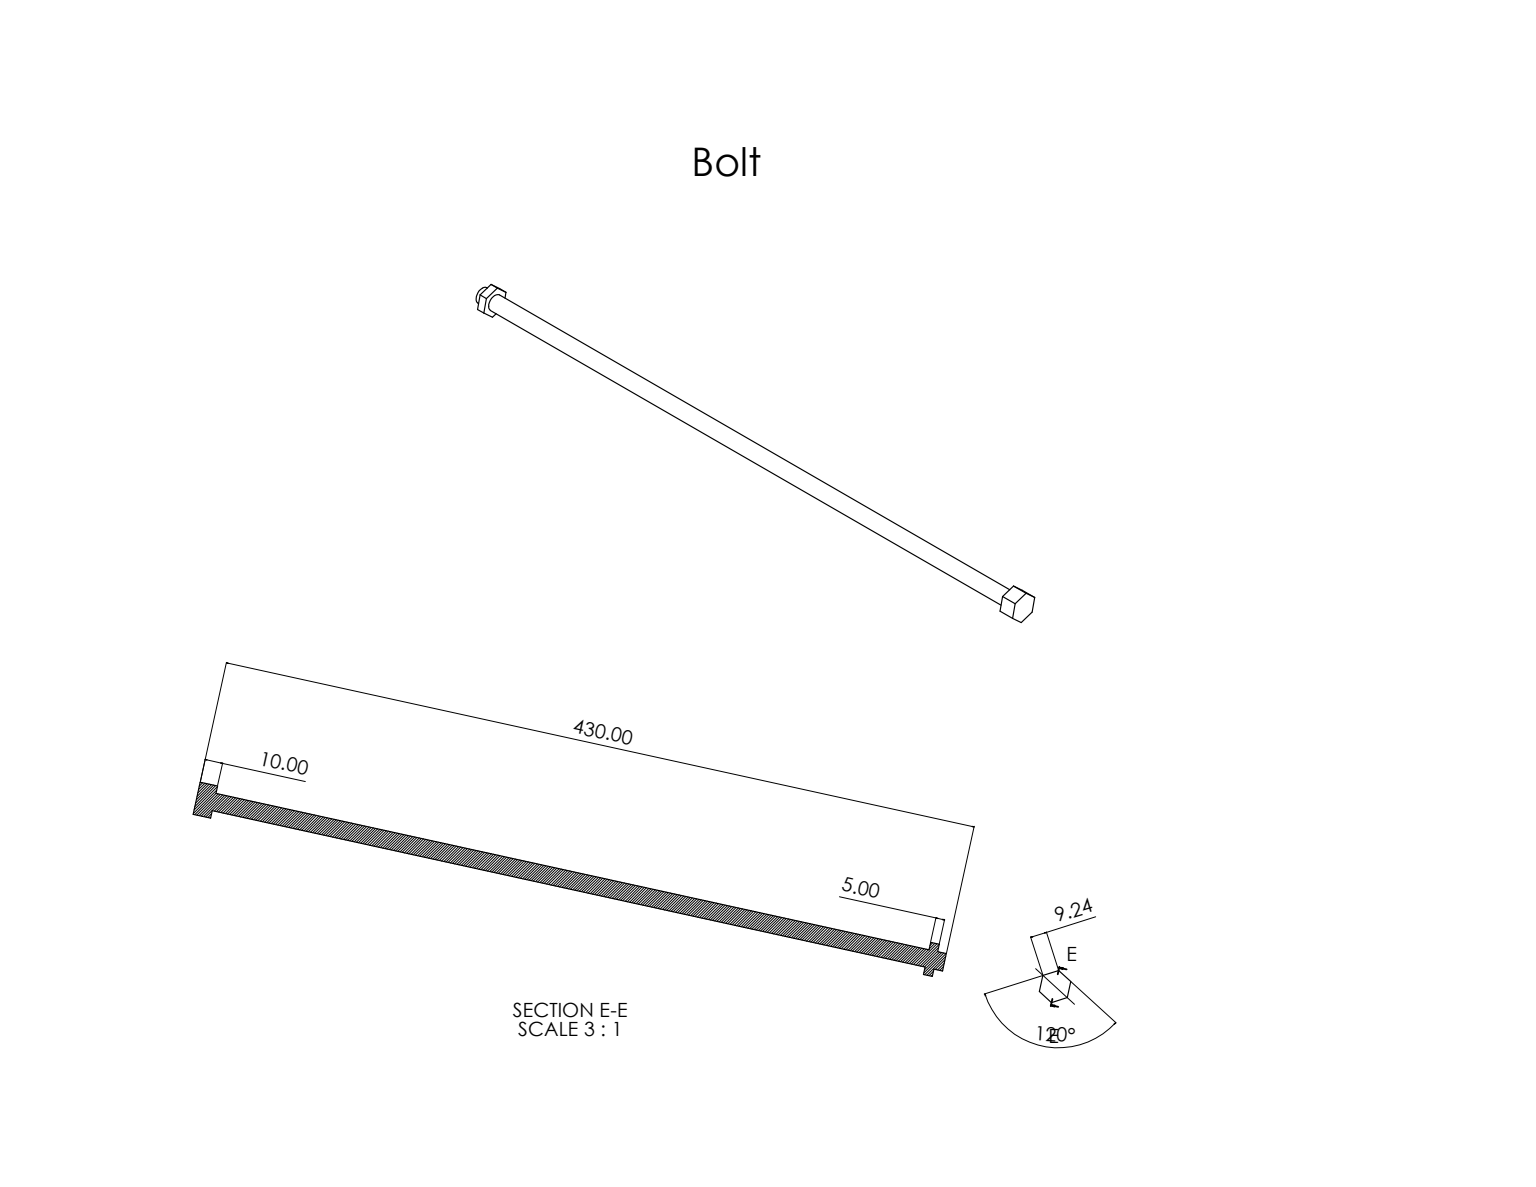
ISO-10303-21;
HEADER;
FILE_DESCRIPTION (('STEP AP214'),
    '1' );
FILE_NAME ('Bolt.step',
    '2026-10-27T19:20:31',
    ( '' ),
    ( '' ),
    'SwSTEP 2.0',
    'SolidWorks 2025',
    '' );
FILE_SCHEMA (( 'AUTOMOTIVE_DESIGN' ));
ENDSEC;

DATA;
#7=DIRECTION ( 'NONE',  ( 0.000000000000000000, 0.000000000000000000, -1.000000000000000000 ) ) ;
#22=DIRECTION ( 'NONE',  ( 0.000000000000000000, 0.000000000000000000, 1.000000000000000000 ) ) ;
#49=EDGE_CURVE ( 'NONE', #17928, #4130, #15424, .T. ) ;
#84=AXIS2_PLACEMENT_3D ( 'NONE', #861, #18677, #15078 ) ;
#112=ORIENTED_EDGE ( 'NONE', *, *, #21174, .F. ) ;
#117=EDGE_CURVE ( 'NONE', #6149, #16510, #26225, .T. ) ;
#141=ADVANCED_FACE ( 'NONE', ( #24347 ), #25952, .T. ) ;
#186=ORIENTED_EDGE ( 'NONE', *, *, #13817, .T. ) ;
#194=DIRECTION ( 'NONE',  ( 0.000000000000000000, -0.9767746502210199466, 0.2142691827715878239 ) ) ;
#196=CARTESIAN_POINT ( 'NONE',  ( 210.0000000000000284, 61.50000000000009948, -66.50000000000005684 ) ) ;
#258=PLANE ( 'NONE',  #2201 ) ;
#310=DIRECTION ( 'NONE',  ( 0.000000000000000000, -0.6739498806388346530, -0.7387770694782699321 ) ) ;
#394=ORIENTED_EDGE ( 'NONE', *, *, #6967, .F. ) ;
#426=( NAMED_UNIT ( * ) SI_UNIT ( $, .STERADIAN. ) SOLID_ANGLE_UNIT ( ) );
#446=DIRECTION ( 'NONE',  ( 0.000000000000000000, 0.000000000000000000, -1.000000000000000000 ) ) ;
#471=CARTESIAN_POINT ( 'NONE',  ( -215.0000000000000284, 69.29737539576900929, -75.30386416458597409 ) ) ;
#528=ORIENTED_EDGE ( 'NONE', *, *, #7839, .T. ) ;
#540=CARTESIAN_POINT ( 'NONE',  ( -215.0000000000000284, 61.50000000000001421, -66.50000000000005684 ) ) ;
#553=CARTESIAN_POINT ( 'NONE',  ( -210.0000000000000284, 72.72568232011437317, -59.67546976104961942 ) ) ;
#556=DIRECTION ( 'NONE',  ( -1.000000000000000000, -1.836970198721030427E-16, 0.000000000000000000 ) ) ;
#568=ORIENTED_EDGE ( 'NONE', *, *, #18157, .T. ) ;
#576=FACE_OUTER_BOUND ( 'NONE', #10089, .T. ) ;
#580=LINE ( 'NONE', #4839, #17878 ) ;
#732=DIRECTION ( 'NONE',  ( 1.000000000000000000, 1.836970198721030181E-16, 0.000000000000000000 ) ) ;
#831=EDGE_LOOP ( 'NONE', ( #23466, #9560, #14259, #11065 ) ) ;
#861=CARTESIAN_POINT ( 'NONE',  ( 200.0000000000000000, 66.50000000000009948, -66.50000000000005684 ) ) ;
#876=LINE ( 'NONE', #6848, #22484 ) ;
#879=CARTESIAN_POINT ( 'NONE',  ( 210.0000000000000284, 69.29737539576909455, -75.30386416458597409 ) ) ;
#902=CARTESIAN_POINT ( 'NONE',  ( 210.0000000000000284, 72.72568232011447265, -59.67546976104962653 ) ) ;
#912=CARTESIAN_POINT ( 'NONE',  ( -210.0000000000000284, 63.70262460423102624, -57.69613583541415380 ) ) ;
#916=VERTEX_POINT ( 'NONE', #14930 ) ;
#964=DIRECTION ( 'NONE',  ( -1.000000000000000000, -1.836970198721030427E-16, 0.000000000000000000 ) ) ;
#1015=ORIENTED_EDGE ( 'NONE', *, *, #8422, .F. ) ;
#1091=DIRECTION ( 'NONE',  ( -1.000000000000000000, -1.836970198721030181E-16, -0.000000000000000000 ) ) ;
#1229=VECTOR ( 'NONE', #17312, 999.9999999999998863 ) ;
#1242=CARTESIAN_POINT ( 'NONE',  ( 210.0000000000000284, 57.47694228411675255, -64.52066607436459833 ) ) ;
#1306=LINE ( 'NONE', #11034, #4996 ) ;
#1348=CARTESIAN_POINT ( 'NONE',  ( -210.0000000000000284, 69.29737539576900929, -75.30386416458597409 ) ) ;
#1465=DIRECTION ( 'NONE',  ( 0.000000000000000000, 0.9767746502210199466, -0.2142691827715878516 ) ) ;
#1540=CARTESIAN_POINT ( 'NONE',  ( 200.0000000000000000, 60.27431767988573341, -73.32453023895050137 ) ) ;
#1585=ORIENTED_EDGE ( 'NONE', *, *, #12200, .F. ) ;
#1664=EDGE_CURVE ( 'NONE', #23424, #6149, #13484, .T. ) ;
#1682=CARTESIAN_POINT ( 'NONE',  ( -210.0000000000000284, 72.72568232011437317, -59.67546976104961942 ) ) ;
#1694=LINE ( 'NONE', #15510, #2299 ) ;
#1718=VECTOR ( 'NONE', #5729, 1000.000000000000000 ) ;
#1774=DIRECTION ( 'NONE',  ( 1.000000000000000000, 1.836970198721030181E-16, 0.000000000000000000 ) ) ;
#1865=DIRECTION ( 'NONE',  ( 3.936061032557164822E-17, -0.2142691827715878794, -0.9767746502210200576 ) ) ;
#1930=ORIENTED_EDGE ( 'NONE', *, *, #13283, .T. ) ;
#1976=PLANE ( 'NONE',  #22060 ) ;
#1992=ORIENTED_EDGE ( 'NONE', *, *, #23543, .T. ) ;
#2117=CARTESIAN_POINT ( 'NONE',  ( 200.0000000000000000, 57.47694228411675255, -64.52066607436459833 ) ) ;
#2201=AXIS2_PLACEMENT_3D ( 'NONE', #2794, #2665, #8636 ) ;
#2220=VECTOR ( 'NONE', #5945, 1000.000000000000000 ) ;
#2299=VECTOR ( 'NONE', #14052, 1000.000000000000000 ) ;
#2341=EDGE_CURVE ( 'NONE', #17934, #4130, #16539, .T. ) ;
#2366=VECTOR ( 'NONE', #194, 1000.000000000000227 ) ;
#2367=VECTOR ( 'NONE', #4874, 1000.000000000000114 ) ;
#2378=ORIENTED_EDGE ( 'NONE', *, *, #17423, .F. ) ;
#2442=DIRECTION ( 'NONE',  ( -1.000000000000000000, -1.836970198721030427E-16, 0.000000000000000000 ) ) ;
#2524=DIRECTION ( 'NONE',  ( 0.000000000000000000, -0.6739498806388345420, -0.7387770694782699321 ) ) ;
#2544=ORIENTED_EDGE ( 'NONE', *, *, #15330, .F. ) ;
#2545=LINE ( 'NONE', #8794, #12997 ) ;
#2567=EDGE_CURVE ( 'NONE', #9742, #21974, #6511, .T. ) ;
#2578=DIRECTION ( 'NONE',  ( -1.000000000000000000, -1.836970198721030181E-16, -0.000000000000000000 ) ) ;
#2595=VERTEX_POINT ( 'NONE', #10778 ) ;
#2601=DIRECTION ( 'NONE',  ( -1.000000000000000000, -1.836970198721030181E-16, -0.000000000000000000 ) ) ;
#2665=DIRECTION ( 'NONE',  ( -1.750717563385751092E-16, 0.9530462522498561739, 0.3028247695821851271 ) ) ;
#2667=DIRECTION ( 'NONE',  ( 0.000000000000000000, 0.6739498806388349861, 0.7387770694782697101 ) ) ;
#2688=ORIENTED_EDGE ( 'NONE', *, *, #11249, .T. ) ;
#2786=CARTESIAN_POINT ( 'NONE',  ( 210.0000000000000284, 66.50000000000009948, -66.50000000000005684 ) ) ;
#2794=CARTESIAN_POINT ( 'NONE',  ( 200.0000000000000000, 75.52305771588345351, -68.47933392563552957 ) ) ;
#2798=CIRCLE ( 'NONE', #6593, 5.000000000000004441 ) ;
#2818=VERTEX_POINT ( 'NONE', #540 ) ;
#2865=DIRECTION ( 'NONE',  ( 0.000000000000000000, 0.6739498806388346530, 0.7387770694782699321 ) ) ;
#2919=DIRECTION ( 'NONE',  ( 1.000000000000000000, 1.836970198721030181E-16, 0.000000000000000000 ) ) ;
#2957=LINE ( 'NONE', #11067, #16649 ) ;
#2993=PRODUCT_DEFINITION_CONTEXT ( 'detailed design', #22452, 'design' ) ;
#3022=AXIS2_PLACEMENT_3D ( 'NONE', #23693, #13325, #5473 ) ;
#3042=CIRCLE ( 'NONE', #25569, 5.000000000000004441 ) ;
#3062=EDGE_CURVE ( 'NONE', #2595, #17934, #24018, .T. ) ;
#3091=CARTESIAN_POINT ( 'NONE',  ( 210.0000000000000284, 66.50000000000009948, -66.50000000000005684 ) ) ;
#3169=CARTESIAN_POINT ( 'NONE',  ( 210.0000000000000284, 75.52305771588345351, -68.47933392563552957 ) ) ;
#3191=CARTESIAN_POINT ( 'NONE',  ( -215.0000000000000284, 66.50000000000001421, -66.50000000000005684 ) ) ;
#3201=VERTEX_POINT ( 'NONE', #22834 ) ;
#3204=VECTOR ( 'NONE', #2442, 1000.000000000000000 ) ;
#3266=EDGE_CURVE ( 'NONE', #24713, #12692, #16837, .T. ) ;
#3267=PLANE ( 'NONE',  #7250 ) ;
#3332=CARTESIAN_POINT ( 'NONE',  ( -210.0000000000000284, 60.27431767988564104, -73.32453023895048716 ) ) ;
#3376=DIRECTION ( 'NONE',  ( -1.357111460130038308E-16, 0.7387770694782700431, -0.6739498806388346530 ) ) ;
#3551=ORIENTED_EDGE ( 'NONE', *, *, #21174, .T. ) ;
#3563=DIRECTION ( 'NONE',  ( 0.000000000000000000, 0.000000000000000000, 1.000000000000000000 ) ) ;
#3630=PLANE ( 'NONE',  #18958 ) ;
#3669=VECTOR ( 'NONE', #5582, 999.9999999999998863 ) ;
#3674=CARTESIAN_POINT ( 'NONE',  ( -215.0000000000000284, 66.50000000000001421, -66.50000000000005684 ) ) ;
#3686=ORIENTED_EDGE ( 'NONE', *, *, #9254, .T. ) ;
#3717=EDGE_LOOP ( 'NONE', ( #394, #9608, #568, #16105 ) ) ;
#3722=CARTESIAN_POINT ( 'NONE',  ( -210.0000000000000284, 69.29737539576900929, -75.30386416458597409 ) ) ;
#3759=ORIENTED_EDGE ( 'NONE', *, *, #19081, .F. ) ;
#3764=AXIS2_PLACEMENT_3D ( 'NONE', #15560, #13566, #13698 ) ;
#3770=PLANE ( 'NONE',  #13222 ) ;
#3826=VERTEX_POINT ( 'NONE', #13413 ) ;
#3852=ORIENTED_EDGE ( 'NONE', *, *, #15330, .T. ) ;
#3870=VECTOR ( 'NONE', #23818, 1000.000000000000000 ) ;
#3879=ADVANCED_FACE ( 'NONE', ( #21791, #7802 ), #23912, .T. ) ;
#3898=CIRCLE ( 'NONE', #17049, 5.000000000000004441 ) ;
#3900=LINE ( 'NONE', #20389, #10244 ) ;
#3902=AXIS2_PLACEMENT_3D ( 'NONE', #12330, #10210, #20458 ) ;
#3961=LINE ( 'NONE', #16045, #2220 ) ;
#3985=ORIENTED_EDGE ( 'NONE', *, *, #21595, .F. ) ;
#4036=PRODUCT_DEFINITION_SHAPE ( 'NONE', 'NONE',  #8176 ) ;
#4096=EDGE_LOOP ( 'NONE', ( #20816, #186 ) ) ;
#4117=AXIS2_PLACEMENT_3D ( 'NONE', #15963, #12247, #18363 ) ;
#4130=VERTEX_POINT ( 'NONE', #26285 ) ;
#4152=PLANE ( 'NONE',  #4117 ) ;
#4172=EDGE_LOOP ( 'NONE', ( #8266, #6834, #3852, #6664 ) ) ;
#4182=CARTESIAN_POINT ( 'NONE',  ( -210.0000000000000284, 66.50000000000001421, -66.50000000000005684 ) ) ;
#4241=DIRECTION ( 'NONE',  ( 0.000000000000000000, -0.6739498806388346530, -0.7387770694782699321 ) ) ;
#4265=VERTEX_POINT ( 'NONE', #10027 ) ;
#4370=CARTESIAN_POINT ( 'NONE',  ( 210.0000000000000284, 71.50000000000009948, -66.50000000000005684 ) ) ;
#4443=EDGE_CURVE ( 'NONE', #916, #3826, #2545, .T. ) ;
#4479=( GEOMETRIC_REPRESENTATION_CONTEXT ( 3 ) GLOBAL_UNCERTAINTY_ASSIGNED_CONTEXT ( ( #21345 ) ) GLOBAL_UNIT_ASSIGNED_CONTEXT ( ( #8933, #24908, #426 ) ) REPRESENTATION_CONTEXT ( 'NONE', 'WORKASPACE' ) );
#4503=CARTESIAN_POINT ( 'NONE',  ( -215.0000000000000284, 72.72568232011437317, -59.67546976104961942 ) ) ;
#4541=EDGE_CURVE ( 'NONE', #916, #15838, #25694, .T. ) ;
#4554=CARTESIAN_POINT ( 'NONE',  ( 200.0000000000000000, 72.72568232011447265, -59.67546976104962653 ) ) ;
#4839=CARTESIAN_POINT ( 'NONE',  ( 200.0000000000000000, 69.29737539576909455, -75.30386416458597409 ) ) ;
#4856=CARTESIAN_POINT ( 'NONE',  ( 200.0000000000000000, 69.29737539576909455, -75.30386416458597409 ) ) ;
#4874=DIRECTION ( 'NONE',  ( 0.000000000000000000, 0.6739498806388345420, 0.7387770694782699321 ) ) ;
#4913=LINE ( 'NONE', #9032, #23004 ) ;
#4996=VECTOR ( 'NONE', #6901, 1000.000000000000000 ) ;
#5018=FACE_OUTER_BOUND ( 'NONE', #24466, .T. ) ;
#5084=ORIENTED_EDGE ( 'NONE', *, *, #17492, .F. ) ;
#5124=CARTESIAN_POINT ( 'NONE',  ( -220.0000000000000284, 61.50000000000001421, -66.50000000000005684 ) ) ;
#5222=CARTESIAN_POINT ( 'NONE',  ( -210.0000000000000284, 57.47694228411666728, -64.52066607436458412 ) ) ;
#5242=FACE_OUTER_BOUND ( 'NONE', #22253, .T. ) ;
#5333=EDGE_CURVE ( 'NONE', #15169, #7956, #11201, .T. ) ;
#5368=CLOSED_SHELL ( 'NONE', ( #17057, #12399, #7002, #21965, #18670, #8007, #25920, #12918, #10358, #5425, #9718, #5494, #21354, #141, #11720, #24847, #22644, #15938, #3879, #8489, #17108 ) ) ;
#5421=VERTEX_POINT ( 'NONE', #10120 ) ;
#5425=ADVANCED_FACE ( 'NONE', ( #9720, #23951 ), #26103, .F. ) ;
#5473=DIRECTION ( 'NONE',  ( 0.000000000000000000, -1.000000000000000000, 0.000000000000000000 ) ) ;
#5494=ADVANCED_FACE ( 'NONE', ( #15822 ), #4152, .T. ) ;
#5582=DIRECTION ( 'NONE',  ( 0.000000000000000000, 0.3028247695821854046, -0.9530462522498561739 ) ) ;
#5588=CARTESIAN_POINT ( 'NONE',  ( -215.0000000000000284, 63.70262460423102624, -57.69613583541415380 ) ) ;
#5651=FACE_BOUND ( 'NONE', #7221, .T. ) ;
#5729=DIRECTION ( 'NONE',  ( -1.000000000000000000, -1.836970198721030427E-16, 0.000000000000000000 ) ) ;
#5839=SHAPE_DEFINITION_REPRESENTATION ( #4036, #9131 ) ;
#5918=CARTESIAN_POINT ( 'NONE',  ( -220.0000000000000284, 66.50000000000001421, -66.50000000000005684 ) ) ;
#5945=DIRECTION ( 'NONE',  ( 0.000000000000000000, -0.9767746502210202797, 0.2142691827715867137 ) ) ;
#6033=DIRECTION ( 'NONE',  ( -1.000000000000000000, 0.000000000000000000, 0.000000000000000000 ) ) ;
#6059=LINE ( 'NONE', #196, #10503 ) ;
#6136=EDGE_LOOP ( 'NONE', ( #20119, #26186, #18384, #23799 ) ) ;
#6149=VERTEX_POINT ( 'NONE', #1242 ) ;
#6232=ORIENTED_EDGE ( 'NONE', *, *, #12307, .F. ) ;
#6236=ORIENTED_EDGE ( 'NONE', *, *, #22005, .T. ) ;
#6341=LINE ( 'NONE', #4370, #17656 ) ;
#6419=DIRECTION ( 'NONE',  ( 1.000000000000000000, 1.836970198721030181E-16, 0.000000000000000000 ) ) ;
#6507=LINE ( 'NONE', #14617, #7093 ) ;
#6511=LINE ( 'NONE', #16891, #19344 ) ;
#6523=EDGE_LOOP ( 'NONE', ( #8127, #13309, #1015, #18412 ) ) ;
#6569=PLANE ( 'NONE',  #21469 ) ;
#6593=AXIS2_PLACEMENT_3D ( 'NONE', #5918, #21748, #15485 ) ;
#6663=ORIENTED_EDGE ( 'NONE', *, *, #13817, .F. ) ;
#6664=ORIENTED_EDGE ( 'NONE', *, *, #7740, .T. ) ;
#6697=EDGE_LOOP ( 'NONE', ( #2378, #25082, #21556, #6663 ) ) ;
#6700=DIRECTION ( 'NONE',  ( -1.357111460130037815E-16, 0.7387770694782699321, -0.6739498806388346530 ) ) ;
#6761=LINE ( 'NONE', #3169, #9504 ) ;
#6797=ORIENTED_EDGE ( 'NONE', *, *, #18157, .F. ) ;
#6834=ORIENTED_EDGE ( 'NONE', *, *, #23543, .F. ) ;
#6848=CARTESIAN_POINT ( 'NONE',  ( 210.0000000000000284, 72.72568232011447265, -59.67546976104962653 ) ) ;
#6891=EDGE_CURVE ( 'NONE', #24783, #6149, #10356, .T. ) ;
#6901=DIRECTION ( 'NONE',  ( 0.000000000000000000, 0.9767746502210202797, -0.2142691827715865471 ) ) ;
#6962=FACE_OUTER_BOUND ( 'NONE', #15182, .T. ) ;
#6967=EDGE_CURVE ( 'NONE', #12692, #10794, #6761, .T. ) ;
#6992=CARTESIAN_POINT ( 'NONE',  ( -210.0000000000000284, 61.50000000000001421, -66.50000000000005684 ) ) ;
#7002=ADVANCED_FACE ( 'NONE', ( #13151 ), #7017, .T. ) ;
#7017=CYLINDRICAL_SURFACE ( 'NONE', #24391, 5.000000000000004441 ) ;
#7093=VECTOR ( 'NONE', #2667, 1000.000000000000000 ) ;
#7111=DIRECTION ( 'NONE',  ( 0.000000000000000000, -0.9767746502210202797, 0.2142691827715867137 ) ) ;
#7189=EDGE_CURVE ( 'NONE', #24779, #10794, #1694, .T. ) ;
#7221=EDGE_LOOP ( 'NONE', ( #14771, #17843 ) ) ;
#7250=AXIS2_PLACEMENT_3D ( 'NONE', #15236, #21492, #13123 ) ;
#7317=CARTESIAN_POINT ( 'NONE',  ( 210.0000000000000284, 66.50000000000009948, -66.50000000000005684 ) ) ;
#7398=CARTESIAN_POINT ( 'NONE',  ( 200.0000000000000000, 75.52305771588345351, -68.47933392563552957 ) ) ;
#7558=ORIENTED_EDGE ( 'NONE', *, *, #19074, .T. ) ;
#7700=LINE ( 'NONE', #5588, #8515 ) ;
#7705=DIRECTION ( 'NONE',  ( 0.000000000000000000, -0.3028247695821854046, 0.9530462522498561739 ) ) ;
#7711=CARTESIAN_POINT ( 'NONE',  ( 200.0000000000000000, -1.836970198721029589E-15, 0.000000000000000000 ) ) ;
#7740=EDGE_CURVE ( 'NONE', #13337, #4265, #20450, .T. ) ;
#7802=FACE_OUTER_BOUND ( 'NONE', #24410, .T. ) ;
#7815=ORIENTED_EDGE ( 'NONE', *, *, #7740, .F. ) ;
#7819=ORIENTED_EDGE ( 'NONE', *, *, #5333, .T. ) ;
#7839=EDGE_CURVE ( 'NONE', #24783, #15800, #22979, .T. ) ;
#7876=DIRECTION ( 'NONE',  ( 1.357111460130037815E-16, -0.7387770694782699321, 0.6739498806388346530 ) ) ;
#7913=DIRECTION ( 'NONE',  ( 0.000000000000000000, 0.3028247695821862928, -0.9530462522498558409 ) ) ;
#7956=VERTEX_POINT ( 'NONE', #6992 ) ;
#7994=CARTESIAN_POINT ( 'NONE',  ( 0.000000000000000000, 0.000000000000000000, 0.000000000000000000 ) ) ;
#8001=ORIENTED_EDGE ( 'NONE', *, *, #18091, .F. ) ;
#8007=ADVANCED_FACE ( 'NONE', ( #5018 ), #3267, .T. ) ;
#8127=ORIENTED_EDGE ( 'NONE', *, *, #20727, .T. ) ;
#8172=CARTESIAN_POINT ( 'NONE',  ( -220.0000000000000284, 75.00000000000000000, 0.000000000000000000 ) ) ;
#8176=PRODUCT_DEFINITION ( 'UNKNOWN', '', #21086, #2993 ) ;
#8266=ORIENTED_EDGE ( 'NONE', *, *, #19899, .F. ) ;
#8293=ORIENTED_EDGE ( 'NONE', *, *, #7839, .F. ) ;
#8299=STYLED_ITEM('',(#26402),#8434);
#8356=EDGE_LOOP ( 'NONE', ( #8973, #11864, #12964, #17976 ) ) ;
#8422=EDGE_CURVE ( 'NONE', #9561, #3201, #2798, .T. ) ;
#8434=MANIFOLD_SOLID_BREP ( 'Boss-Extrude6', #5368 ) ;
#8464=CARTESIAN_POINT ( 'NONE',  ( -210.0000000000000284, 63.70262460423102624, -57.69613583541415380 ) ) ;
#8489=ADVANCED_FACE ( 'NONE', ( #12426 ), #6569, .F. ) ;
#8515=VECTOR ( 'NONE', #19432, 1000.000000000000114 ) ;
#8530=SHAPE_REPRESENTATION_RELATIONSHIP ( 'NONE' , 'NONE' ,  #9131, #22943 ) ;
#8542=AXIS2_PLACEMENT_3D ( 'NONE', #4182, #6033, #15997 ) ;
#8636=DIRECTION ( 'NONE',  ( 0.000000000000000000, -0.3028247695821851271, 0.9530462522498561739 ) ) ;
#8659=ORIENTED_EDGE ( 'NONE', *, *, #10442, .T. ) ;
#8774=AXIS2_PLACEMENT_3D ( 'NONE', #3091, #1091, #9199 ) ;
#8794=CARTESIAN_POINT ( 'NONE',  ( -210.0000000000000284, 69.29737539576900929, -75.30386416458597409 ) ) ;
#8933=( LENGTH_UNIT ( ) NAMED_UNIT ( * ) SI_UNIT ( .MILLI., .METRE. ) );
#8939=DIRECTION ( 'NONE',  ( 0.000000000000000000, 0.3028247695821862928, -0.9530462522498558409 ) ) ;
#8970=LINE ( 'NONE', #24954, #10285 ) ;
#8973=ORIENTED_EDGE ( 'NONE', *, *, #22005, .F. ) ;
#9030=DIRECTION ( 'NONE',  ( 0.000000000000000000, -0.3028247695821851271, 0.9530462522498561739 ) ) ;
#9032=CARTESIAN_POINT ( 'NONE',  ( 200.0000000000000000, 60.27431767988573341, -73.32453023895050137 ) ) ;
#9121=DIRECTION ( 'NONE',  ( 0.000000000000000000, 0.3028247695821854046, -0.9530462522498561739 ) ) ;
#9131=SHAPE_REPRESENTATION ( 'Bolt', ( #21058 ), #4479 ) ;
#9199=DIRECTION ( 'NONE',  ( 0.000000000000000000, -1.000000000000000000, 0.000000000000000000 ) ) ;
#9254=EDGE_CURVE ( 'NONE', #3826, #5421, #12430, .T. ) ;
#9430=CARTESIAN_POINT ( 'NONE',  ( 200.0000000000000000, 75.52305771588345351, -68.47933392563552957 ) ) ;
#9438=AXIS2_PLACEMENT_3D ( 'NONE', #19539, #17537, #15664 ) ;
#9446=PLANE ( 'NONE',  #25585 ) ;
#9504=VECTOR ( 'NONE', #9030, 1000.000000000000114 ) ;
#9510=DIRECTION ( 'NONE',  ( -1.000000000000000000, 0.000000000000000000, 0.000000000000000000 ) ) ;
#9522=DIRECTION ( 'NONE',  ( 0.000000000000000000, -1.000000000000000000, 0.000000000000000000 ) ) ;
#9526=ORIENTED_EDGE ( 'NONE', *, *, #4443, .F. ) ;
#9560=ORIENTED_EDGE ( 'NONE', *, *, #18585, .F. ) ;
#9561=VERTEX_POINT ( 'NONE', #5124 ) ;
#9564=ORIENTED_EDGE ( 'NONE', *, *, #23937, .F. ) ;
#9608=ORIENTED_EDGE ( 'NONE', *, *, #19074, .F. ) ;
#9682=FACE_OUTER_BOUND ( 'NONE', #19932, .T. ) ;
#9718=ADVANCED_FACE ( 'NONE', ( #5242 ), #3630, .T. ) ;
#9720=FACE_BOUND ( 'NONE', #22871, .T. ) ;
#9742=VERTEX_POINT ( 'NONE', #23715 ) ;
#9817=CARTESIAN_POINT ( 'NONE',  ( -215.0000000000000284, 9.184850993605151889E-16, 0.000000000000000000 ) ) ;
#9929=CARTESIAN_POINT ( 'NONE',  ( -210.0000000000000284, 57.47694228411666728, -64.52066607436458412 ) ) ;
#9968=CARTESIAN_POINT ( 'NONE',  ( 210.0000000000000284, 57.47694228411675255, -64.52066607436459833 ) ) ;
#9993=ORIENTED_EDGE ( 'NONE', *, *, #11249, .F. ) ;
#10027=CARTESIAN_POINT ( 'NONE',  ( -215.0000000000000284, 63.70262460423102624, -57.69613583541415380 ) ) ;
#10082=CARTESIAN_POINT ( 'NONE',  ( -210.0000000000000284, 63.70262460423102624, -57.69613583541415380 ) ) ;
#10089=EDGE_LOOP ( 'NONE', ( #9993, #24065, #21429, #22083 ) ) ;
#10120=CARTESIAN_POINT ( 'NONE',  ( -215.0000000000000284, 60.27431767988564104, -73.32453023895048716 ) ) ;
#10210=DIRECTION ( 'NONE',  ( -1.000000000000000000, -1.836970198721030181E-16, -0.000000000000000000 ) ) ;
#10244=VECTOR ( 'NONE', #24109, 1000.000000000000000 ) ;
#10285=VECTOR ( 'NONE', #732, 1000.000000000000000 ) ;
#10306=ORIENTED_EDGE ( 'NONE', *, *, #18007, .F. ) ;
#10356=LINE ( 'NONE', #2117, #20571 ) ;
#10358=ADVANCED_FACE ( 'NONE', ( #576 ), #22924, .T. ) ;
#10387=DIRECTION ( 'NONE',  ( 0.000000000000000000, -0.3028247695821862928, 0.9530462522498558409 ) ) ;
#10395=ORIENTED_EDGE ( 'NONE', *, *, #20727, .F. ) ;
#10442=EDGE_CURVE ( 'NONE', #5421, #14022, #21823, .T. ) ;
#10446=VECTOR ( 'NONE', #15432, 1000.000000000000227 ) ;
#10475=EDGE_CURVE ( 'NONE', #15838, #18515, #11700, .T. ) ;
#10503=VECTOR ( 'NONE', #2601, 1000.000000000000000 ) ;
#10648=DIRECTION ( 'NONE',  ( 0.000000000000000000, 0.6739498806388345420, 0.7387770694782699321 ) ) ;
#10688=DIRECTION ( 'NONE',  ( 1.000000000000000000, 0.000000000000000000, 0.000000000000000000 ) ) ;
#10778=CARTESIAN_POINT ( 'NONE',  ( -210.0000000000000284, 72.72568232011437317, -59.67546976104961942 ) ) ;
#10792=FACE_OUTER_BOUND ( 'NONE', #14421, .T. ) ;
#10794=VERTEX_POINT ( 'NONE', #902 ) ;
#10893=LINE ( 'NONE', #912, #22531 ) ;
#10935=ORIENTED_EDGE ( 'NONE', *, *, #117, .F. ) ;
#10939=ORIENTED_EDGE ( 'NONE', *, *, #3266, .T. ) ;
#11028=ORIENTED_EDGE ( 'NONE', *, *, #13296, .F. ) ;
#11034=CARTESIAN_POINT ( 'NONE',  ( 200.0000000000000000, 60.27431767988573341, -73.32453023895050137 ) ) ;
#11065=ORIENTED_EDGE ( 'NONE', *, *, #6891, .T. ) ;
#11067=CARTESIAN_POINT ( 'NONE',  ( -210.0000000000000284, 72.72568232011437317, -59.67546976104961942 ) ) ;
#11201=LINE ( 'NONE', #15318, #25742 ) ;
#11249=EDGE_CURVE ( 'NONE', #10794, #23424, #876, .T. ) ;
#11272=DIRECTION ( 'NONE',  ( 0.000000000000000000, -1.000000000000000000, 0.000000000000000000 ) ) ;
#11294=AXIS2_PLACEMENT_3D ( 'NONE', #9817, #25796, #3563 ) ;
#11300=DIRECTION ( 'NONE',  ( 0.000000000000000000, -1.000000000000000000, 0.000000000000000000 ) ) ;
#11429=CARTESIAN_POINT ( 'NONE',  ( -215.0000000000000284, 72.72568232011437317, -59.67546976104961942 ) ) ;
#11609=PLANE ( 'NONE',  #24611 ) ;
#11628=CARTESIAN_POINT ( 'NONE',  ( -210.0000000000000284, 60.27431767988564104, -73.32453023895048716 ) ) ;
#11700=LINE ( 'NONE', #15310, #1229 ) ;
#11720=ADVANCED_FACE ( 'NONE', ( #23477 ), #11609, .T. ) ;
#11749=CARTESIAN_POINT ( 'NONE',  ( 200.0000000000000000, 63.70262460423112572, -57.69613583541415380 ) ) ;
#11864=ORIENTED_EDGE ( 'NONE', *, *, #2341, .F. ) ;
#11951=LINE ( 'NONE', #9430, #15777 ) ;
#12128=( GEOMETRIC_REPRESENTATION_CONTEXT ( 3 ) GLOBAL_UNCERTAINTY_ASSIGNED_CONTEXT ( ( #17779 ) ) GLOBAL_UNIT_ASSIGNED_CONTEXT ( ( #18682, #16685, #14424 ) ) REPRESENTATION_CONTEXT ( 'NONE', 'WORKASPACE' ) );
#12200=EDGE_CURVE ( 'NONE', #18548, #17450, #19195, .T. ) ;
#12247=DIRECTION ( 'NONE',  ( 1.357111460130037815E-16, -0.7387770694782697101, 0.6739498806388349861 ) ) ;
#12307=EDGE_CURVE ( 'NONE', #15838, #5421, #19317, .T. ) ;
#12330=CARTESIAN_POINT ( 'NONE',  ( -220.0000000000000284, 66.50000000000001421, -66.50000000000005684 ) ) ;
#12399=ADVANCED_FACE ( 'NONE', ( #15569 ), #19569, .T. ) ;
#12405=VECTOR ( 'NONE', #22187, 1000.000000000000000 ) ;
#12426=FACE_OUTER_BOUND ( 'NONE', #4096, .T. ) ;
#12430=LINE ( 'NONE', #471, #2366 ) ;
#12489=CARTESIAN_POINT ( 'NONE',  ( -215.0000000000000284, 75.52305771588336825, -68.47933392563552957 ) ) ;
#12653=PLANE ( 'NONE',  #16150 ) ;
#12692=VERTEX_POINT ( 'NONE', #20902 ) ;
#12748=PRODUCT ( 'Bolt', 'Bolt', '', ( #26078 ) ) ;
#12751=ORIENTED_EDGE ( 'NONE', *, *, #4541, .T. ) ;
#12796=ORIENTED_EDGE ( 'NONE', *, *, #2341, .T. ) ;
#12918=ADVANCED_FACE ( 'NONE', ( #24531 ), #3770, .T. ) ;
#12964=ORIENTED_EDGE ( 'NONE', *, *, #18007, .T. ) ;
#12997=VECTOR ( 'NONE', #556, 1000.000000000000000 ) ;
#13048=CARTESIAN_POINT ( 'NONE',  ( 200.0000000000000000, 61.50000000000009948, -66.50000000000005684 ) ) ;
#13075=EDGE_CURVE ( 'NONE', #17450, #7956, #24274, .T. ) ;
#13123=DIRECTION ( 'NONE',  ( 0.000000000000000000, 0.9767746502210202797, -0.2142691827715865471 ) ) ;
#13151=FACE_OUTER_BOUND ( 'NONE', #20391, .T. ) ;
#13162=CARTESIAN_POINT ( 'NONE',  ( 210.0000000000000284, 60.27431767988573341, -73.32453023895050137 ) ) ;
#13222=AXIS2_PLACEMENT_3D ( 'NONE', #17985, #7876, #310 ) ;
#13283=EDGE_CURVE ( 'NONE', #9742, #24713, #580, .T. ) ;
#13296=EDGE_CURVE ( 'NONE', #15169, #18548, #3042, .T. ) ;
#13309=ORIENTED_EDGE ( 'NONE', *, *, #17423, .T. ) ;
#13325=DIRECTION ( 'NONE',  ( -1.000000000000000000, -1.836970198721030181E-16, -0.000000000000000000 ) ) ;
#13337=VERTEX_POINT ( 'NONE', #14537 ) ;
#13347=CARTESIAN_POINT ( 'NONE',  ( 210.0000000000000284, 66.50000000000009948, -66.50000000000005684 ) ) ;
#13406=VECTOR ( 'NONE', #7913, 1000.000000000000000 ) ;
#13413=CARTESIAN_POINT ( 'NONE',  ( -215.0000000000000284, 69.29737539576900929, -75.30386416458597409 ) ) ;
#13484=LINE ( 'NONE', #15355, #24884 ) ;
#13566=DIRECTION ( 'NONE',  ( -3.936061032557143868E-17, 0.2142691827715866859, 0.9767746502210202797 ) ) ;
#13595=DIRECTION ( 'NONE',  ( -1.836970198721030181E-16, 1.000000000000000000, 0.000000000000000000 ) ) ;
#13661=AXIS2_PLACEMENT_3D ( 'NONE', #4856, #6700, #2865 ) ;
#13698=DIRECTION ( 'NONE',  ( 0.000000000000000000, -0.9767746502210202797, 0.2142691827715866859 ) ) ;
#13807=ORIENTED_EDGE ( 'NONE', *, *, #3062, .F. ) ;
#13817=EDGE_CURVE ( 'NONE', #3201, #9561, #15350, .T. ) ;
#13853=VECTOR ( 'NONE', #4241, 1000.000000000000000 ) ;
#13894=CARTESIAN_POINT ( 'NONE',  ( -210.0000000000000284, 1.836970198721030378E-15, 0.000000000000000000 ) ) ;
#13944=EDGE_LOOP ( 'NONE', ( #6797, #17804, #17174, #8293, #5084, #3759 ) ) ;
#14022=VERTEX_POINT ( 'NONE', #23498 ) ;
#14052=DIRECTION ( 'NONE',  ( 1.000000000000000000, 1.836970198721030181E-16, 0.000000000000000000 ) ) ;
#14055=EDGE_LOOP ( 'NONE', ( #20338, #6232, #20318, #1992 ) ) ;
#14083=ORIENTED_EDGE ( 'NONE', *, *, #13296, .T. ) ;
#14222=LINE ( 'NONE', #20485, #14517 ) ;
#14236=DIRECTION ( 'NONE',  ( 1.000000000000000000, 0.000000000000000000, 0.000000000000000000 ) ) ;
#14259=ORIENTED_EDGE ( 'NONE', *, *, #17492, .T. ) ;
#14378=PLANE ( 'NONE',  #19943 ) ;
#14421=EDGE_LOOP ( 'NONE', ( #19810, #112, #22551, #12796 ) ) ;
#14424=( NAMED_UNIT ( * ) SI_UNIT ( $, .STERADIAN. ) SOLID_ANGLE_UNIT ( ) );
#14517=VECTOR ( 'NONE', #18348, 1000.000000000000000 ) ;
#14537=CARTESIAN_POINT ( 'NONE',  ( -210.0000000000000284, 63.70262460423102624, -57.69613583541415380 ) ) ;
#14617=CARTESIAN_POINT ( 'NONE',  ( -210.0000000000000284, 57.47694228411666728, -64.52066607436458412 ) ) ;
#14740=VERTEX_POINT ( 'NONE', #11749 ) ;
#14771=ORIENTED_EDGE ( 'NONE', *, *, #18178, .T. ) ;
#14815=EDGE_LOOP ( 'NONE', ( #10395, #8001 ) ) ;
#14902=DIRECTION ( 'NONE',  ( 0.000000000000000000, -0.6739498806388345420, -0.7387770694782699321 ) ) ;
#14930=CARTESIAN_POINT ( 'NONE',  ( -210.0000000000000284, 69.29737539576900929, -75.30386416458597409 ) ) ;
#14931=CARTESIAN_POINT ( 'NONE',  ( 200.0000000000000000, 66.50000000000009948, -66.50000000000005684 ) ) ;
#15078=DIRECTION ( 'NONE',  ( 0.000000000000000000, 0.000000000000000000, -1.000000000000000000 ) ) ;
#15169=VERTEX_POINT ( 'NONE', #13048 ) ;
#15176=ORIENTED_EDGE ( 'NONE', *, *, #6891, .F. ) ;
#15182=EDGE_LOOP ( 'NONE', ( #17536, #19138, #23271, #7558 ) ) ;
#15188=FACE_OUTER_BOUND ( 'NONE', #6523, .T. ) ;
#15204=ORIENTED_EDGE ( 'NONE', *, *, #1664, .T. ) ;
#15236=CARTESIAN_POINT ( 'NONE',  ( 200.0000000000000000, 60.27431767988573341, -73.32453023895050137 ) ) ;
#15298=VERTEX_POINT ( 'NONE', #24026 ) ;
#15310=CARTESIAN_POINT ( 'NONE',  ( -210.0000000000000284, 60.27431767988564104, -73.32453023895048716 ) ) ;
#15318=CARTESIAN_POINT ( 'NONE',  ( 210.0000000000000284, 61.50000000000009948, -66.50000000000005684 ) ) ;
#15330=EDGE_CURVE ( 'NONE', #18515, #13337, #6507, .T. ) ;
#15350=CIRCLE ( 'NONE', #3902, 5.000000000000004441 ) ;
#15355=CARTESIAN_POINT ( 'NONE',  ( 210.0000000000000284, 63.70262460423112572, -57.69613583541415380 ) ) ;
#15424=LINE ( 'NONE', #11429, #21106 ) ;
#15427=DIRECTION ( 'NONE',  ( 1.750717563385751339E-16, -0.9530462522498560629, -0.3028247695821853491 ) ) ;
#15431=DIRECTION ( 'NONE',  ( -1.000000000000000000, -1.836970198721030181E-16, -0.000000000000000000 ) ) ;
#15432=DIRECTION ( 'NONE',  ( 0.000000000000000000, -0.9767746502210199466, 0.2142691827715878239 ) ) ;
#15469=DIRECTION ( 'NONE',  ( 0.000000000000000000, 0.6739498806388345420, 0.7387770694782699321 ) ) ;
#15485=DIRECTION ( 'NONE',  ( 0.000000000000000000, 1.000000000000000000, 0.000000000000000000 ) ) ;
#15510=CARTESIAN_POINT ( 'NONE',  ( 200.0000000000000000, 72.72568232011447265, -59.67546976104962653 ) ) ;
#15552=EDGE_CURVE ( 'NONE', #15800, #9742, #1306, .T. ) ;
#15560=CARTESIAN_POINT ( 'NONE',  ( 200.0000000000000000, 72.72568232011447265, -59.67546976104962653 ) ) ;
#15569=FACE_OUTER_BOUND ( 'NONE', #6136, .T. ) ;
#15618=PLANE ( 'NONE',  #23262 ) ;
#15664=DIRECTION ( 'NONE',  ( 0.000000000000000000, 0.000000000000000000, 1.000000000000000000 ) ) ;
#15669=ORIENTED_EDGE ( 'NONE', *, *, #12307, .T. ) ;
#15777=VECTOR ( 'NONE', #23790, 1000.000000000000114 ) ;
#15800=VERTEX_POINT ( 'NONE', #1540 ) ;
#15822=FACE_OUTER_BOUND ( 'NONE', #4172, .T. ) ;
#15838=VERTEX_POINT ( 'NONE', #11628 ) ;
#15938=ADVANCED_FACE ( 'NONE', ( #5651, #20157 ), #15618, .F. ) ;
#15963=CARTESIAN_POINT ( 'NONE',  ( -210.0000000000000284, 57.47694228411666728, -64.52066607436458412 ) ) ;
#15977=DIRECTION ( 'NONE',  ( 1.000000000000000000, 0.000000000000000000, 0.000000000000000000 ) ) ;
#15997=DIRECTION ( 'NONE',  ( 0.000000000000000000, 0.000000000000000000, 1.000000000000000000 ) ) ;
#16045=CARTESIAN_POINT ( 'NONE',  ( 200.0000000000000000, 72.72568232011447265, -59.67546976104962653 ) ) ;
#16105=ORIENTED_EDGE ( 'NONE', *, *, #7189, .T. ) ;
#16141=EDGE_CURVE ( 'NONE', #2818, #9561, #6059, .T. ) ;
#16150=AXIS2_PLACEMENT_3D ( 'NONE', #21041, #19043, #20779 ) ;
#16286=DIRECTION ( 'NONE',  ( 1.000000000000000000, 1.836970198721030181E-16, 0.000000000000000000 ) ) ;
#16324=CARTESIAN_POINT ( 'NONE',  ( -210.0000000000000284, 71.50000000000002842, -66.50000000000005684 ) ) ;
#16510=VERTEX_POINT ( 'NONE', #13162 ) ;
#16539=LINE ( 'NONE', #22805, #3204 ) ;
#16649=VECTOR ( 'NONE', #964, 1000.000000000000000 ) ;
#16685=( NAMED_UNIT ( * ) PLANE_ANGLE_UNIT ( ) SI_UNIT ( $, .RADIAN. ) );
#16741=ORIENTED_EDGE ( 'NONE', *, *, #117, .T. ) ;
#16837=LINE ( 'NONE', #879, #2367 ) ;
#16891=CARTESIAN_POINT ( 'NONE',  ( 200.0000000000000000, 69.29737539576909455, -75.30386416458597409 ) ) ;
#16942=ORIENTED_EDGE ( 'NONE', *, *, #4541, .F. ) ;
#16945=PLANE ( 'NONE',  #13661 ) ;
#16975=ORIENTED_EDGE ( 'NONE', *, *, #21595, .T. ) ;
#17049=AXIS2_PLACEMENT_3D ( 'NONE', #3674, #25903, #9522 ) ;
#17057=ADVANCED_FACE ( 'NONE', ( #15188 ), #23314, .T. ) ;
#17108=ADVANCED_FACE ( 'NONE', ( #17431 ), #25571, .T. ) ;
#17174=ORIENTED_EDGE ( 'NONE', *, *, #15552, .F. ) ;
#17263=DIRECTION ( 'NONE',  ( -1.000000000000000000, -1.836970198721030181E-16, -0.000000000000000000 ) ) ;
#17309=CARTESIAN_POINT ( 'NONE',  ( 210.0000000000000284, 63.70262460423112572, -57.69613583541415380 ) ) ;
#17312=DIRECTION ( 'NONE',  ( 0.000000000000000000, -0.3028247695821854046, 0.9530462522498561739 ) ) ;
#17418=ORIENTED_EDGE ( 'NONE', *, *, #20550, .F. ) ;
#17423=EDGE_CURVE ( 'NONE', #15298, #3201, #6341, .T. ) ;
#17431=FACE_OUTER_BOUND ( 'NONE', #6697, .T. ) ;
#17450=VERTEX_POINT ( 'NONE', #16324 ) ;
#17492=EDGE_CURVE ( 'NONE', #14740, #24783, #24452, .T. ) ;
#17536=ORIENTED_EDGE ( 'NONE', *, *, #3266, .F. ) ;
#17537=DIRECTION ( 'NONE',  ( -1.000000000000000000, 0.000000000000000000, 0.000000000000000000 ) ) ;
#17656=VECTOR ( 'NONE', #26058, 1000.000000000000000 ) ;
#17779=UNCERTAINTY_MEASURE_WITH_UNIT (LENGTH_MEASURE( 1.000000000000000082E-05 ), #18682, 'distance_accuracy_value', 'NONE');
#17804=ORIENTED_EDGE ( 'NONE', *, *, #2567, .F. ) ;
#17843=ORIENTED_EDGE ( 'NONE', *, *, #13075, .T. ) ;
#17878=VECTOR ( 'NONE', #6419, 1000.000000000000000 ) ;
#17909=ORIENTED_EDGE ( 'NONE', *, *, #10475, .F. ) ;
#17928=VERTEX_POINT ( 'NONE', #4503 ) ;
#17934=VERTEX_POINT ( 'NONE', #18726 ) ;
#17976=ORIENTED_EDGE ( 'NONE', *, *, #4443, .T. ) ;
#17985=CARTESIAN_POINT ( 'NONE',  ( 200.0000000000000000, 63.70262460423112572, -57.69613583541415380 ) ) ;
#18007=EDGE_CURVE ( 'NONE', #17934, #916, #18905, .T. ) ;
#18091=EDGE_CURVE ( 'NONE', #15298, #2818, #21747, .T. ) ;
#18157=EDGE_CURVE ( 'NONE', #21974, #24779, #11951, .T. ) ;
#18178=EDGE_CURVE ( 'NONE', #7956, #17450, #20935, .T. ) ;
#18186=DIRECTION ( 'NONE',  ( -3.936061032557131542E-17, 0.2142691827715860198, 0.9767746502210203907 ) ) ;
#18308=VECTOR ( 'NONE', #2578, 1000.000000000000000 ) ;
#18348=DIRECTION ( 'NONE',  ( 0.000000000000000000, 0.9767746502210202797, -0.2142691827715865471 ) ) ;
#18363=DIRECTION ( 'NONE',  ( 0.000000000000000000, -0.6739498806388349861, -0.7387770694782697101 ) ) ;
#18379=ORIENTED_EDGE ( 'NONE', *, *, #23231, .T. ) ;
#18384=ORIENTED_EDGE ( 'NONE', *, *, #18178, .F. ) ;
#18412=ORIENTED_EDGE ( 'NONE', *, *, #16141, .F. ) ;
#18413=ORIENTED_EDGE ( 'NONE', *, *, #15552, .T. ) ;
#18515=VERTEX_POINT ( 'NONE', #9929 ) ;
#18548=VERTEX_POINT ( 'NONE', #20577 ) ;
#18555=AXIS2_PLACEMENT_3D ( 'NONE', #7711, #14236, #7 ) ;
#18582=VECTOR ( 'NONE', #20319, 1000.000000000000000 ) ;
#18585=EDGE_CURVE ( 'NONE', #14740, #23424, #8970, .T. ) ;
#18670=ADVANCED_FACE ( 'NONE', ( #6962 ), #16945, .T. ) ;
#18677=DIRECTION ( 'NONE',  ( 1.000000000000000000, 0.000000000000000000, 0.000000000000000000 ) ) ;
#18679=ORIENTED_EDGE ( 'NONE', *, *, #18722, .T. ) ;
#18682=( LENGTH_UNIT ( ) NAMED_UNIT ( * ) SI_UNIT ( .MILLI., .METRE. ) );
#18722=EDGE_CURVE ( 'NONE', #18548, #15169, #19633, .T. ) ;
#18726=CARTESIAN_POINT ( 'NONE',  ( -210.0000000000000284, 75.52305771588336825, -68.47933392563552957 ) ) ;
#18774=CARTESIAN_POINT ( 'NONE',  ( 210.0000000000000284, 69.29737539576909455, -75.30386416458597409 ) ) ;
#18874=DIRECTION ( 'NONE',  ( 1.000000000000000000, 1.836970198721030181E-16, 0.000000000000000000 ) ) ;
#18905=LINE ( 'NONE', #25296, #22809 ) ;
#18958=AXIS2_PLACEMENT_3D ( 'NONE', #13347, #1774, #13595 ) ;
#19006=DIRECTION ( 'NONE',  ( 0.000000000000000000, 0.9767746502210203907, -0.2142691827715860198 ) ) ;
#19043=DIRECTION ( 'NONE',  ( 1.750717563385750846E-16, -0.9530462522498561739, -0.3028247695821854046 ) ) ;
#19074=EDGE_CURVE ( 'NONE', #21974, #12692, #25652, .T. ) ;
#19081=EDGE_CURVE ( 'NONE', #24779, #14740, #3961, .T. ) ;
#19109=CARTESIAN_POINT ( 'NONE',  ( 200.0000000000000000, 57.47694228411675255, -64.52066607436459833 ) ) ;
#19110=APPLICATION_CONTEXT ( 'automotive_design' ) ;
#19138=ORIENTED_EDGE ( 'NONE', *, *, #13283, .F. ) ;
#19195=LINE ( 'NONE', #23325, #18308 ) ;
#19302=FACE_OUTER_BOUND ( 'NONE', #14055, .T. ) ;
#19317=LINE ( 'NONE', #25581, #3870 ) ;
#19344=VECTOR ( 'NONE', #10648, 1000.000000000000114 ) ;
#19430=DIRECTION ( 'NONE',  ( 0.000000000000000000, 0.3028247695821853491, -0.9530462522498560629 ) ) ;
#19432=DIRECTION ( 'NONE',  ( 0.000000000000000000, 0.9767746502210203907, -0.2142691827715860198 ) ) ;
#19539=CARTESIAN_POINT ( 'NONE',  ( -210.0000000000000284, 66.50000000000001421, -66.50000000000005684 ) ) ;
#19569=CYLINDRICAL_SURFACE ( 'NONE', #3022, 5.000000000000004441 ) ;
#19605=DIRECTION ( 'NONE',  ( 0.000000000000000000, -0.6739498806388346530, -0.7387770694782699321 ) ) ;
#19633=CIRCLE ( 'NONE', #84, 5.000000000000004441 ) ;
#19810=ORIENTED_EDGE ( 'NONE', *, *, #49, .F. ) ;
#19822=CARTESIAN_POINT ( 'NONE',  ( -215.0000000000000284, 60.27431767988564104, -73.32453023895048716 ) ) ;
#19899=EDGE_CURVE ( 'NONE', #14022, #4265, #3900, .T. ) ;
#19932=EDGE_LOOP ( 'NONE', ( #20087, #7815, #20821, #3551 ) ) ;
#19943=AXIS2_PLACEMENT_3D ( 'NONE', #553, #20907, #10387 ) ;
#20087=ORIENTED_EDGE ( 'NONE', *, *, #23231, .F. ) ;
#20119=ORIENTED_EDGE ( 'NONE', *, *, #18722, .F. ) ;
#20157=FACE_OUTER_BOUND ( 'NONE', #26223, .T. ) ;
#20318=ORIENTED_EDGE ( 'NONE', *, *, #10475, .T. ) ;
#20319=DIRECTION ( 'NONE',  ( -1.000000000000000000, -1.836970198721030427E-16, 0.000000000000000000 ) ) ;
#20338=ORIENTED_EDGE ( 'NONE', *, *, #10442, .F. ) ;
#20389=CARTESIAN_POINT ( 'NONE',  ( -215.0000000000000284, 57.47694228411666728, -64.52066607436458412 ) ) ;
#20391=EDGE_LOOP ( 'NONE', ( #1585, #11028, #7819, #25649 ) ) ;
#20420=EDGE_LOOP ( 'NONE', ( #21983, #9526, #12751, #15669 ) ) ;
#20450=LINE ( 'NONE', #8464, #18582 ) ;
#20458=DIRECTION ( 'NONE',  ( 0.000000000000000000, 1.000000000000000000, 0.000000000000000000 ) ) ;
#20485=CARTESIAN_POINT ( 'NONE',  ( 210.0000000000000284, 60.27431767988573341, -73.32453023895050137 ) ) ;
#20550=EDGE_CURVE ( 'NONE', #15800, #16510, #4913, .T. ) ;
#20555=DIRECTION ( 'NONE',  ( -1.836970198721030181E-16, 1.000000000000000000, 0.000000000000000000 ) ) ;
#20571=VECTOR ( 'NONE', #18874, 1000.000000000000000 ) ;
#20577=CARTESIAN_POINT ( 'NONE',  ( 200.0000000000000000, 71.50000000000009948, -66.50000000000005684 ) ) ;
#20727=EDGE_CURVE ( 'NONE', #2818, #15298, #3898, .T. ) ;
#20754=LINE ( 'NONE', #12489, #22597 ) ;
#20779=DIRECTION ( 'NONE',  ( 0.000000000000000000, 0.3028247695821854046, -0.9530462522498561739 ) ) ;
#20816=ORIENTED_EDGE ( 'NONE', *, *, #8422, .T. ) ;
#20821=ORIENTED_EDGE ( 'NONE', *, *, #23937, .T. ) ;
#20902=CARTESIAN_POINT ( 'NONE',  ( 210.0000000000000284, 75.52305771588345351, -68.47933392563552957 ) ) ;
#20907=DIRECTION ( 'NONE',  ( -1.750717563385750846E-16, 0.9530462522498558409, 0.3028247695821862928 ) ) ;
#20935=CIRCLE ( 'NONE', #9438, 5.000000000000004441 ) ;
#21038=CARTESIAN_POINT ( 'NONE',  ( 200.0000000000000000, 57.47694228411675255, -64.52066607436459833 ) ) ;
#21041=CARTESIAN_POINT ( 'NONE',  ( 200.0000000000000000, 57.47694228411675255, -64.52066607436459833 ) ) ;
#21058=AXIS2_PLACEMENT_3D ( 'NONE', #7994, #22, #15977 ) ;
#21086=PRODUCT_DEFINITION_FORMATION_WITH_SPECIFIED_SOURCE ( 'ANY', '', #12748, .NOT_KNOWN. ) ;
#21106=VECTOR ( 'NONE', #8939, 1000.000000000000000 ) ;
#21174=EDGE_CURVE ( 'NONE', #2595, #17928, #2957, .T. ) ;
#21345=UNCERTAINTY_MEASURE_WITH_UNIT (LENGTH_MEASURE( 1.000000000000000082E-05 ), #8933, 'distance_accuracy_value', 'NONE');
#21354=ADVANCED_FACE ( 'NONE', ( #19302 ), #9446, .T. ) ;
#21429=ORIENTED_EDGE ( 'NONE', *, *, #19081, .T. ) ;
#21469=AXIS2_PLACEMENT_3D ( 'NONE', #8172, #16286, #20555 ) ;
#21475=CARTESIAN_POINT ( 'NONE',  ( -210.0000000000000284, 75.52305771588336825, -68.47933392563552957 ) ) ;
#21492=DIRECTION ( 'NONE',  ( 3.936061032557140787E-17, -0.2142691827715865471, -0.9767746502210202797 ) ) ;
#21556=ORIENTED_EDGE ( 'NONE', *, *, #16141, .T. ) ;
#21595=EDGE_CURVE ( 'NONE', #16510, #24713, #14222, .T. ) ;
#21747=CIRCLE ( 'NONE', #24323, 5.000000000000004441 ) ;
#21748=DIRECTION ( 'NONE',  ( -1.000000000000000000, -1.836970198721030181E-16, -0.000000000000000000 ) ) ;
#21791=FACE_BOUND ( 'NONE', #14815, .T. ) ;
#21823=LINE ( 'NONE', #19822, #25041 ) ;
#21965=ADVANCED_FACE ( 'NONE', ( #23020 ), #258, .T. ) ;
#21974=VERTEX_POINT ( 'NONE', #25015 ) ;
#21983=ORIENTED_EDGE ( 'NONE', *, *, #9254, .F. ) ;
#22005=EDGE_CURVE ( 'NONE', #4130, #3826, #20754, .T. ) ;
#22060=AXIS2_PLACEMENT_3D ( 'NONE', #10082, #18186, #26337 ) ;
#22083=ORIENTED_EDGE ( 'NONE', *, *, #18585, .T. ) ;
#22187=DIRECTION ( 'NONE',  ( 1.000000000000000000, 1.836970198721030181E-16, 0.000000000000000000 ) ) ;
#22214=EDGE_LOOP ( 'NONE', ( #10935, #15176, #528, #23925 ) ) ;
#22253=EDGE_LOOP ( 'NONE', ( #22974, #2688, #15204, #16741, #16975, #10939 ) ) ;
#22368=AXIS2_PLACEMENT_3D ( 'NONE', #7317, #15431, #23558 ) ;
#22452=APPLICATION_CONTEXT ( 'automotive_design' ) ;
#22461=CARTESIAN_POINT ( 'NONE',  ( 200.0000000000000000, 63.70262460423112572, -57.69613583541415380 ) ) ;
#22484=VECTOR ( 'NONE', #7111, 1000.000000000000000 ) ;
#22531=VECTOR ( 'NONE', #19006, 1000.000000000000114 ) ;
#22551=ORIENTED_EDGE ( 'NONE', *, *, #3062, .T. ) ;
#22597=VECTOR ( 'NONE', #2524, 1000.000000000000114 ) ;
#22644=ADVANCED_FACE ( 'NONE', ( #9682 ), #1976, .T. ) ;
#22805=CARTESIAN_POINT ( 'NONE',  ( -210.0000000000000284, 75.52305771588336825, -68.47933392563552957 ) ) ;
#22809=VECTOR ( 'NONE', #14902, 1000.000000000000114 ) ;
#22834=CARTESIAN_POINT ( 'NONE',  ( -220.0000000000000284, 71.50000000000002842, -66.50000000000005684 ) ) ;
#22871=EDGE_LOOP ( 'NONE', ( #14083, #18679 ) ) ;
#22924=PLANE ( 'NONE',  #3764 ) ;
#22943=ADVANCED_BREP_SHAPE_REPRESENTATION ( '', ( #8434, #21058 ), #4479 ) ;
#22974=ORIENTED_EDGE ( 'NONE', *, *, #6967, .T. ) ;
#22979=LINE ( 'NONE', #19109, #25545 ) ;
#23004=VECTOR ( 'NONE', #2919, 1000.000000000000000 ) ;
#23020=FACE_OUTER_BOUND ( 'NONE', #3717, .T. ) ;
#23172=FACE_OUTER_BOUND ( 'NONE', #22214, .T. ) ;
#23231=EDGE_CURVE ( 'NONE', #4265, #17928, #7700, .T. ) ;
#23262=AXIS2_PLACEMENT_3D ( 'NONE', #13894, #9510, #23741 ) ;
#23271=ORIENTED_EDGE ( 'NONE', *, *, #2567, .T. ) ;
#23314=CYLINDRICAL_SURFACE ( 'NONE', #8774, 5.000000000000004441 ) ;
#23325=CARTESIAN_POINT ( 'NONE',  ( 210.0000000000000284, 71.50000000000009948, -66.50000000000005684 ) ) ;
#23424=VERTEX_POINT ( 'NONE', #17309 ) ;
#23466=ORIENTED_EDGE ( 'NONE', *, *, #1664, .F. ) ;
#23477=FACE_OUTER_BOUND ( 'NONE', #8356, .T. ) ;
#23498=CARTESIAN_POINT ( 'NONE',  ( -215.0000000000000284, 57.47694228411666728, -64.52066607436458412 ) ) ;
#23543=EDGE_CURVE ( 'NONE', #18515, #14022, #25455, .T. ) ;
#23558=DIRECTION ( 'NONE',  ( 0.000000000000000000, -1.000000000000000000, 0.000000000000000000 ) ) ;
#23593=MECHANICAL_DESIGN_GEOMETRIC_PRESENTATION_REPRESENTATION('',(#8299),#12128);
#23693=CARTESIAN_POINT ( 'NONE',  ( 210.0000000000000284, 66.50000000000009948, -66.50000000000005684 ) ) ;
#23715=CARTESIAN_POINT ( 'NONE',  ( 200.0000000000000000, 69.29737539576909455, -75.30386416458597409 ) ) ;
#23741=DIRECTION ( 'NONE',  ( 0.000000000000000000, 0.000000000000000000, 1.000000000000000000 ) ) ;
#23790=DIRECTION ( 'NONE',  ( 0.000000000000000000, -0.3028247695821851271, 0.9530462522498561739 ) ) ;
#23799=ORIENTED_EDGE ( 'NONE', *, *, #5333, .F. ) ;
#23818=DIRECTION ( 'NONE',  ( -1.000000000000000000, -1.836970198721030427E-16, 0.000000000000000000 ) ) ;
#23912=PLANE ( 'NONE',  #11294 ) ;
#23925=ORIENTED_EDGE ( 'NONE', *, *, #20550, .T. ) ;
#23937=EDGE_CURVE ( 'NONE', #13337, #2595, #10893, .T. ) ;
#23951=FACE_OUTER_BOUND ( 'NONE', #13944, .T. ) ;
#24018=LINE ( 'NONE', #1682, #13406 ) ;
#24026=CARTESIAN_POINT ( 'NONE',  ( -215.0000000000000284, 71.50000000000002842, -66.50000000000005684 ) ) ;
#24065=ORIENTED_EDGE ( 'NONE', *, *, #7189, .F. ) ;
#24109=DIRECTION ( 'NONE',  ( 0.000000000000000000, 0.6739498806388349861, 0.7387770694782697101 ) ) ;
#24274=CIRCLE ( 'NONE', #8542, 5.000000000000004441 ) ;
#24323=AXIS2_PLACEMENT_3D ( 'NONE', #3191, #25426, #11300 ) ;
#24347=FACE_OUTER_BOUND ( 'NONE', #20420, .T. ) ;
#24391=AXIS2_PLACEMENT_3D ( 'NONE', #2786, #17263, #11272 ) ;
#24410=EDGE_LOOP ( 'NONE', ( #25210, #18379, #24507, #6236, #3686, #8659 ) ) ;
#24452=LINE ( 'NONE', #22461, #13853 ) ;
#24466=EDGE_LOOP ( 'NONE', ( #3985, #17418, #18413, #1930 ) ) ;
#24507=ORIENTED_EDGE ( 'NONE', *, *, #49, .T. ) ;
#24531=FACE_OUTER_BOUND ( 'NONE', #831, .T. ) ;
#24611=AXIS2_PLACEMENT_3D ( 'NONE', #21475, #3376, #15469 ) ;
#24713=VERTEX_POINT ( 'NONE', #18774 ) ;
#24779=VERTEX_POINT ( 'NONE', #4554 ) ;
#24783=VERTEX_POINT ( 'NONE', #21038 ) ;
#24847=ADVANCED_FACE ( 'NONE', ( #10792 ), #14378, .T. ) ;
#24884=VECTOR ( 'NONE', #19605, 1000.000000000000000 ) ;
#24908=( NAMED_UNIT ( * ) PLANE_ANGLE_UNIT ( ) SI_UNIT ( $, .RADIAN. ) );
#24932=AXIS2_PLACEMENT_3D ( 'NONE', #3722, #1865, #1465 ) ;
#24954=CARTESIAN_POINT ( 'NONE',  ( 200.0000000000000000, 63.70262460423112572, -57.69613583541415380 ) ) ;
#25015=CARTESIAN_POINT ( 'NONE',  ( 200.0000000000000000, 75.52305771588345351, -68.47933392563552957 ) ) ;
#25041=VECTOR ( 'NONE', #7705, 999.9999999999998863 ) ;
#25082=ORIENTED_EDGE ( 'NONE', *, *, #18091, .T. ) ;
#25210=ORIENTED_EDGE ( 'NONE', *, *, #19899, .T. ) ;
#25296=CARTESIAN_POINT ( 'NONE',  ( -210.0000000000000284, 75.52305771588336825, -68.47933392563552957 ) ) ;
#25426=DIRECTION ( 'NONE',  ( -1.000000000000000000, -1.836970198721030181E-16, 0.000000000000000000 ) ) ;
#25455=LINE ( 'NONE', #5222, #1718 ) ;
#25545=VECTOR ( 'NONE', #9121, 999.9999999999998863 ) ;
#25569=AXIS2_PLACEMENT_3D ( 'NONE', #14931, #10688, #446 ) ;
#25571=CYLINDRICAL_SURFACE ( 'NONE', #22368, 5.000000000000004441 ) ;
#25581=CARTESIAN_POINT ( 'NONE',  ( -210.0000000000000284, 60.27431767988564104, -73.32453023895048716 ) ) ;
#25585=AXIS2_PLACEMENT_3D ( 'NONE', #3332, #15427, #19430 ) ;
#25649=ORIENTED_EDGE ( 'NONE', *, *, #13075, .F. ) ;
#25652=LINE ( 'NONE', #7398, #12405 ) ;
#25694=LINE ( 'NONE', #1348, #10446 ) ;
#25742=VECTOR ( 'NONE', #25971, 1000.000000000000000 ) ;
#25796=DIRECTION ( 'NONE',  ( -1.000000000000000000, 0.000000000000000000, 0.000000000000000000 ) ) ;
#25903=DIRECTION ( 'NONE',  ( -1.000000000000000000, -1.836970198721030181E-16, 0.000000000000000000 ) ) ;
#25920=ADVANCED_FACE ( 'NONE', ( #23172 ), #12653, .T. ) ;
#25952=PLANE ( 'NONE',  #24932 ) ;
#25971=DIRECTION ( 'NONE',  ( -1.000000000000000000, -1.836970198721030181E-16, -0.000000000000000000 ) ) ;
#26058=DIRECTION ( 'NONE',  ( -1.000000000000000000, -1.836970198721030181E-16, -0.000000000000000000 ) ) ;
#26078=PRODUCT_CONTEXT ( 'NONE', #19110, 'mechanical' ) ;
#26103=PLANE ( 'NONE',  #18555 ) ;
#26186=ORIENTED_EDGE ( 'NONE', *, *, #12200, .T. ) ;
#26223=EDGE_LOOP ( 'NONE', ( #2544, #17909, #16942, #10306, #13807, #9564 ) ) ;
#26225=LINE ( 'NONE', #9968, #3669 ) ;
#26285=CARTESIAN_POINT ( 'NONE',  ( -215.0000000000000284, 75.52305771588336825, -68.47933392563552957 ) ) ;
#26337=DIRECTION ( 'NONE',  ( 0.000000000000000000, -0.9767746502210203907, 0.2142691827715860198 ) ) ;
#26396=COLOUR_RGB('Black',0.12,0.14,0.17);
#26397=FILL_AREA_STYLE_COLOUR('',#26396);
#26398=FILL_AREA_STYLE('',(#26397));
#26399=SURFACE_STYLE_FILL_AREA(#26398);
#26400=SURFACE_SIDE_STYLE('',(#26399));
#26401=SURFACE_STYLE_USAGE(.BOTH.,#26400);
#26402=PRESENTATION_STYLE_ASSIGNMENT((#26401));
ENDSEC;
END-ISO-10303-21;
